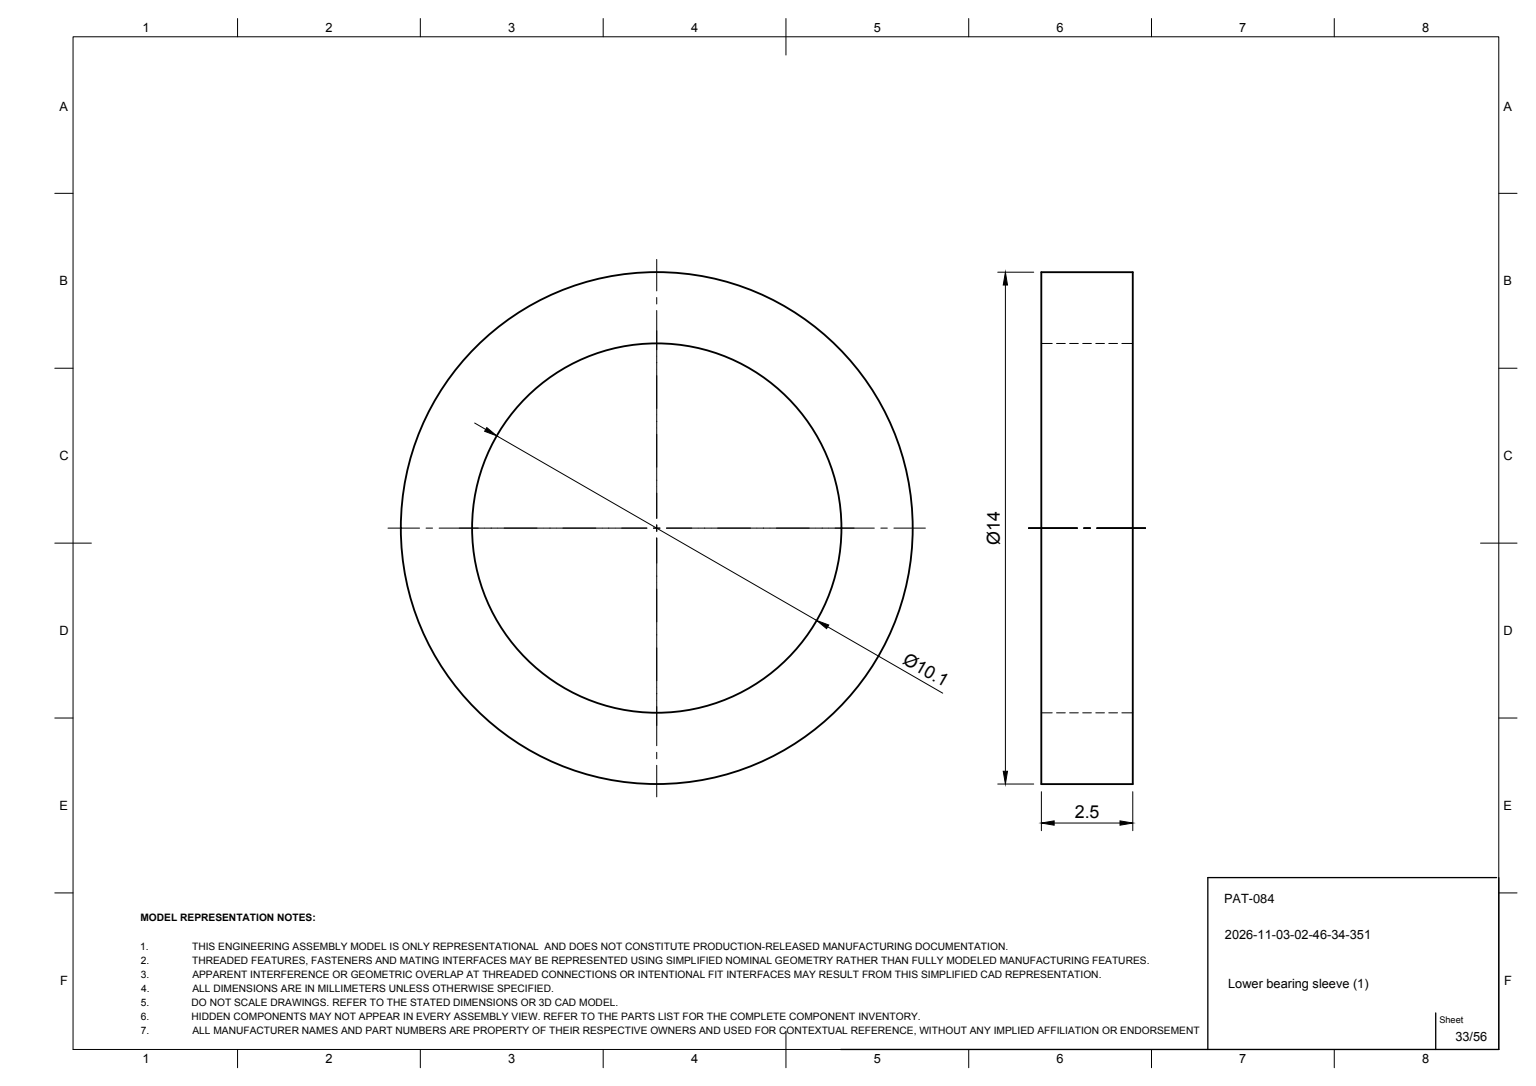
ISO-10303-21;
HEADER;
/* Generated by software containing ST-Developer
 * from STEP Tools, Inc. (www.steptools.com) 
 */

FILE_DESCRIPTION(
/* description */ ('Quick-return (Whitworth) mechanism'),
/* implementation_level */ '2;1');

FILE_NAME(
/* name */ 'Lower bearing sleeve (1).step',
/* time_stamp */ '2026-10-28T03:25:57-07:00',
/* author */ (''),
/* organization */ (''),
/* preprocessor_version */ 'ST-DEVELOPER v20.2',
/* originating_system */ 'Autodesk Translation Framework v15.17.0.0',
/* authorisation */ '');

FILE_SCHEMA (('AUTOMOTIVE_DESIGN { 1 0 10303 214 3 1 1 }'));
ENDSEC;

DATA;
#10=MECHANICAL_DESIGN_GEOMETRIC_PRESENTATION_REPRESENTATION('',(#521),#14878);
#425=SHAPE_REPRESENTATION_RELATIONSHIP('SRR','None',#15096,#469);
#469=ADVANCED_BREP_SHAPE_REPRESENTATION('',(#572),#14853);
#521=STYLED_ITEM('',(#15406),#572);
#572=MANIFOLD_SOLID_BREP('Body1',#7876);
#731=FACE_BOUND('',#1942,.T.);
#732=FACE_BOUND('',#1944,.T.);
#922=PLANE('',#9014);
#923=PLANE('',#9015);
#1333=FACE_OUTER_BOUND('',#1939,.T.);
#1334=FACE_OUTER_BOUND('',#1940,.T.);
#1335=FACE_OUTER_BOUND('',#1941,.T.);
#1336=FACE_OUTER_BOUND('',#1943,.T.);
#1939=EDGE_LOOP('',(#6448,#6449,#6450,#6451));
#1940=EDGE_LOOP('',(#6452,#6453,#6454,#6455));
#1941=EDGE_LOOP('',(#6456));
#1942=EDGE_LOOP('',(#6457));
#1943=EDGE_LOOP('',(#6458));
#1944=EDGE_LOOP('',(#6459));
#2428=LINE('',#13803,#2951);
#2429=LINE('',#13809,#2952);
#2951=VECTOR('',#10907,0.505);
#2952=VECTOR('',#10914,0.7);
#3520=CIRCLE('',#9009,0.505);
#3521=CIRCLE('',#9010,0.505);
#3522=CIRCLE('',#9012,0.7);
#3523=CIRCLE('',#9013,0.7);
#4036=VERTEX_POINT('',#13800);
#4037=VERTEX_POINT('',#13802);
#4038=VERTEX_POINT('',#13806);
#4039=VERTEX_POINT('',#13808);
#4881=EDGE_CURVE('',#4036,#4036,#3520,.T.);
#4882=EDGE_CURVE('',#4036,#4037,#2428,.T.);
#4883=EDGE_CURVE('',#4037,#4037,#3521,.T.);
#4884=EDGE_CURVE('',#4038,#4038,#3522,.T.);
#4885=EDGE_CURVE('',#4038,#4039,#2429,.T.);
#4886=EDGE_CURVE('',#4039,#4039,#3523,.T.);
#6448=ORIENTED_EDGE('',*,*,#4881,.F.);
#6449=ORIENTED_EDGE('',*,*,#4882,.T.);
#6450=ORIENTED_EDGE('',*,*,#4883,.T.);
#6451=ORIENTED_EDGE('',*,*,#4882,.F.);
#6452=ORIENTED_EDGE('',*,*,#4884,.F.);
#6453=ORIENTED_EDGE('',*,*,#4885,.T.);
#6454=ORIENTED_EDGE('',*,*,#4886,.T.);
#6455=ORIENTED_EDGE('',*,*,#4885,.F.);
#6456=ORIENTED_EDGE('',*,*,#4884,.T.);
#6457=ORIENTED_EDGE('',*,*,#4881,.T.);
#6458=ORIENTED_EDGE('',*,*,#4886,.F.);
#6459=ORIENTED_EDGE('',*,*,#4883,.F.);
#7330=CYLINDRICAL_SURFACE('',#9008,0.505);
#7331=CYLINDRICAL_SURFACE('',#9011,0.7);
#7664=ADVANCED_FACE('',(#1333),#7330,.F.);
#7665=ADVANCED_FACE('',(#1334),#7331,.T.);
#7666=ADVANCED_FACE('',(#1335,#731),#922,.T.);
#7667=ADVANCED_FACE('',(#1336,#732),#923,.F.);
#7876=CLOSED_SHELL('',(#7664,#7665,#7666,#7667));
#9007=AXIS2_PLACEMENT_3D('',#13798,#10901,#10902);
#9008=AXIS2_PLACEMENT_3D('',#13799,#10903,#10904);
#9009=AXIS2_PLACEMENT_3D('',#13801,#10905,#10906);
#9010=AXIS2_PLACEMENT_3D('',#13804,#10908,#10909);
#9011=AXIS2_PLACEMENT_3D('',#13805,#10910,#10911);
#9012=AXIS2_PLACEMENT_3D('',#13807,#10912,#10913);
#9013=AXIS2_PLACEMENT_3D('',#13810,#10915,#10916);
#9014=AXIS2_PLACEMENT_3D('',#13811,#10917,#10918);
#9015=AXIS2_PLACEMENT_3D('',#13812,#10919,#10920);
#10901=DIRECTION('axis',(0.,0.,1.));
#10902=DIRECTION('refdir',(1.,0.,0.));
#10903=DIRECTION('center_axis',(0.,0.,1.));
#10904=DIRECTION('ref_axis',(1.,0.,0.));
#10905=DIRECTION('center_axis',(0.,0.,-1.));
#10906=DIRECTION('ref_axis',(1.,0.,0.));
#10907=DIRECTION('',(0.,0.,-1.));
#10908=DIRECTION('center_axis',(0.,0.,-1.));
#10909=DIRECTION('ref_axis',(1.,0.,0.));
#10910=DIRECTION('center_axis',(0.,0.,1.));
#10911=DIRECTION('ref_axis',(1.,0.,0.));
#10912=DIRECTION('center_axis',(0.,0.,1.));
#10913=DIRECTION('ref_axis',(1.,0.,0.));
#10914=DIRECTION('',(0.,0.,-1.));
#10915=DIRECTION('center_axis',(0.,0.,1.));
#10916=DIRECTION('ref_axis',(1.,0.,0.));
#10917=DIRECTION('center_axis',(0.,0.,1.));
#10918=DIRECTION('ref_axis',(1.,0.,0.));
#10919=DIRECTION('center_axis',(0.,0.,1.));
#10920=DIRECTION('ref_axis',(1.,0.,0.));
#13798=CARTESIAN_POINT('',(0.,0.,0.));
#13799=CARTESIAN_POINT('Origin',(0.,0.,1.8));
#13800=CARTESIAN_POINT('',(-0.505,-6.18446633569413E-17,2.05));
#13801=CARTESIAN_POINT('Origin',(0.,0.,2.05));
#13802=CARTESIAN_POINT('',(-0.505,-6.18446633569413E-17,1.8));
#13803=CARTESIAN_POINT('',(-0.505,-6.18446633569413E-17,1.8));
#13804=CARTESIAN_POINT('Origin',(0.,0.,1.8));
#13805=CARTESIAN_POINT('Origin',(0.,0.,1.8));
#13806=CARTESIAN_POINT('',(-0.7,-8.57252759403147E-17,2.05));
#13807=CARTESIAN_POINT('Origin',(0.,0.,2.05));
#13808=CARTESIAN_POINT('',(-0.7,-8.57252759403147E-17,1.8));
#13809=CARTESIAN_POINT('',(-0.7,-8.57252759403147E-17,1.8));
#13810=CARTESIAN_POINT('Origin',(0.,0.,1.8));
#13811=CARTESIAN_POINT('Origin',(0.,0.,2.05));
#13812=CARTESIAN_POINT('Origin',(0.,0.,1.8));
#14799=UNCERTAINTY_MEASURE_WITH_UNIT(LENGTH_MEASURE(0.001),#14879,
'DISTANCE_ACCURACY_VALUE',
'Maximum model space distance between geometric entities at asserted c
onnectivities');
#14824=UNCERTAINTY_MEASURE_WITH_UNIT(LENGTH_MEASURE(0.001),#14879,
'DISTANCE_ACCURACY_VALUE',
'Maximum model space distance between geometric entities at asserted c
onnectivities');
#14853=(
GEOMETRIC_REPRESENTATION_CONTEXT(3)
GLOBAL_UNCERTAINTY_ASSIGNED_CONTEXT((#14799))
GLOBAL_UNIT_ASSIGNED_CONTEXT((#14879,#14881,#14882))
REPRESENTATION_CONTEXT('','3D')
);
#14878=(
GEOMETRIC_REPRESENTATION_CONTEXT(3)
GLOBAL_UNCERTAINTY_ASSIGNED_CONTEXT((#14824))
GLOBAL_UNIT_ASSIGNED_CONTEXT((#14879,#14881,#14882))
REPRESENTATION_CONTEXT('','3D')
);
#14879=(
LENGTH_UNIT()
NAMED_UNIT(*)
SI_UNIT(.CENTI.,.METRE.)
);
#14881=(
NAMED_UNIT(*)
PLANE_ANGLE_UNIT()
SI_UNIT($,.RADIAN.)
);
#14882=(
NAMED_UNIT(*)
SI_UNIT($,.STERADIAN.)
SOLID_ANGLE_UNIT()
);
#14911=SHAPE_DEFINITION_REPRESENTATION(#14969,#15096);
#14969=PRODUCT_DEFINITION_SHAPE('',$,#15150);
#15096=SHAPE_REPRESENTATION('',(#9007),#14853);
#15121=PRODUCT_DEFINITION_CONTEXT('part definition',#15282,'design');
#15150=PRODUCT_DEFINITION('Lower bearing sleeve (1)',
'Lower bearing sleeve (1)',#15203,#15121);
#15203=PRODUCT_DEFINITION_FORMATION('',$,#15312);
#15282=APPLICATION_CONTEXT(
'Core Data for Automotive Mechanical Design Process');
#15283=PRODUCT_CONTEXT('part definition',#15282,'mechanical');
#15312=PRODUCT('Lower bearing sleeve (1)','Lower bearing sleeve (1)',
'Lower bearing sleeve (1)',(#15283));
#15400=COLOUR_RGB('Grey',0.48,0.52,0.57);
#15401=FILL_AREA_STYLE_COLOUR('',#15400);
#15402=FILL_AREA_STYLE('',(#15401));
#15403=SURFACE_STYLE_FILL_AREA(#15402);
#15404=SURFACE_SIDE_STYLE('',(#15403));
#15405=SURFACE_STYLE_USAGE(.BOTH.,#15404);
#15406=PRESENTATION_STYLE_ASSIGNMENT((#15405));
ENDSEC;
END-ISO-10303-21;
